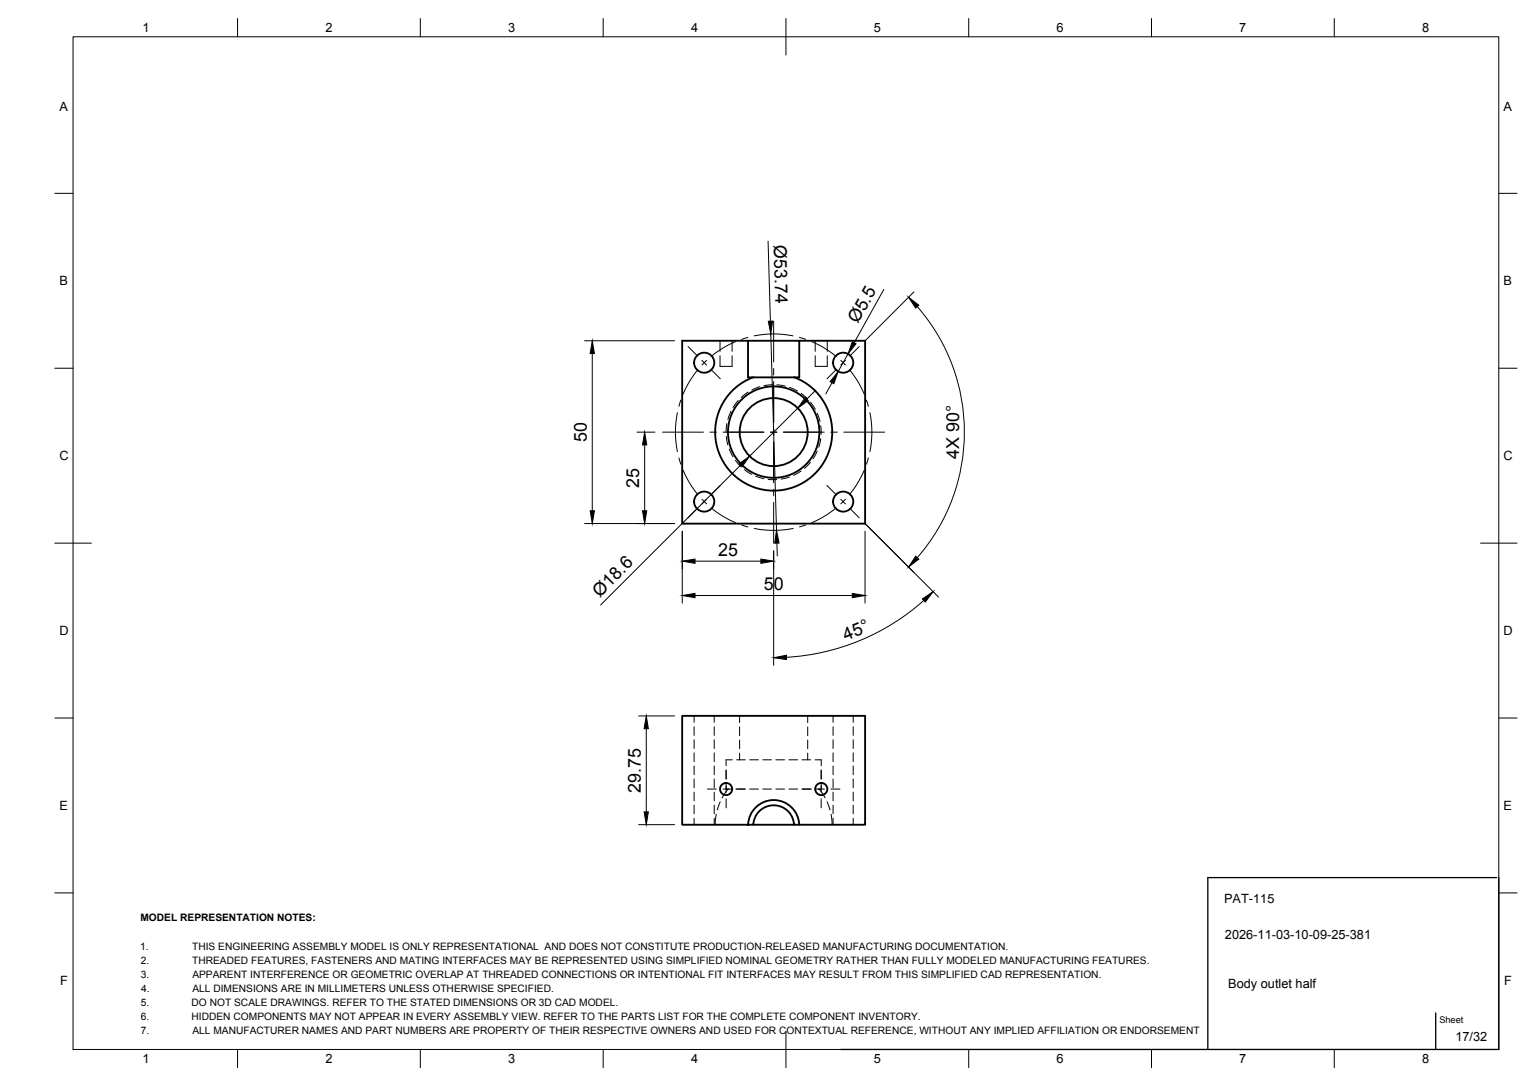
ISO-10303-21;
HEADER;
/* Generated by software containing ST-Developer
 * from STEP Tools, Inc. (www.steptools.com) 
 */

FILE_DESCRIPTION(
/* description */ ('Union bypass pipe loop'),
/* implementation_level */ '2;1');

FILE_NAME(
/* name */ 'Body outlet half.step',
/* time_stamp */ '2026-10-27T21:00:29-07:00',
/* author */ (''),
/* organization */ (''),
/* preprocessor_version */ 'ST-DEVELOPER v20.2',
/* originating_system */ 'Autodesk Translation Framework v15.17.0.0',
/* authorisation */ '');

FILE_SCHEMA (('AUTOMOTIVE_DESIGN { 1 0 10303 214 3 1 1 }'));
ENDSEC;

DATA;
#10=MECHANICAL_DESIGN_GEOMETRIC_PRESENTATION_REPRESENTATION('',(#446),#10095);
#382=SHAPE_REPRESENTATION_RELATIONSHIP('SRR','None',#10251,#414);
#414=ADVANCED_BREP_SHAPE_REPRESENTATION('',(#478),#10063);
#446=STYLED_ITEM('',(#10479),#478);
#478=MANIFOLD_SOLID_BREP('Body1',#5517);
#506=SPHERICAL_SURFACE('',#5987,1.6);
#525=FACE_BOUND('',#1213,.T.);
#526=FACE_BOUND('',#1214,.T.);
#527=FACE_BOUND('',#1218,.T.);
#528=FACE_BOUND('',#1220,.T.);
#529=FACE_BOUND('',#1222,.T.);
#530=FACE_BOUND('',#1224,.T.);
#531=FACE_BOUND('',#1225,.T.);
#532=FACE_BOUND('',#1226,.T.);
#533=FACE_BOUND('',#1227,.T.);
#534=FACE_BOUND('',#1228,.T.);
#535=FACE_BOUND('',#1231,.T.);
#536=FACE_BOUND('',#1232,.T.);
#537=FACE_BOUND('',#1233,.T.);
#538=FACE_BOUND('',#1234,.T.);
#646=PLANE('',#5955);
#647=PLANE('',#5959);
#648=PLANE('',#5975);
#649=PLANE('',#5977);
#650=PLANE('',#5984);
#651=PLANE('',#5985);
#652=PLANE('',#5989);
#653=PLANE('',#5990);
#654=PLANE('',#5991);
#655=PLANE('',#5992);
#656=PLANE('',#5993);
#856=FACE_OUTER_BOUND('',#1202,.T.);
#857=FACE_OUTER_BOUND('',#1203,.T.);
#858=FACE_OUTER_BOUND('',#1204,.T.);
#859=FACE_OUTER_BOUND('',#1205,.T.);
#860=FACE_OUTER_BOUND('',#1206,.T.);
#861=FACE_OUTER_BOUND('',#1207,.T.);
#862=FACE_OUTER_BOUND('',#1208,.T.);
#863=FACE_OUTER_BOUND('',#1209,.T.);
#864=FACE_OUTER_BOUND('',#1210,.T.);
#865=FACE_OUTER_BOUND('',#1211,.T.);
#866=FACE_OUTER_BOUND('',#1212,.T.);
#867=FACE_OUTER_BOUND('',#1215,.T.);
#868=FACE_OUTER_BOUND('',#1216,.T.);
#869=FACE_OUTER_BOUND('',#1217,.T.);
#870=FACE_OUTER_BOUND('',#1219,.T.);
#871=FACE_OUTER_BOUND('',#1221,.T.);
#872=FACE_OUTER_BOUND('',#1223,.T.);
#873=FACE_OUTER_BOUND('',#1229,.T.);
#874=FACE_OUTER_BOUND('',#1230,.T.);
#875=FACE_OUTER_BOUND('',#1235,.T.);
#876=FACE_OUTER_BOUND('',#1236,.T.);
#1202=EDGE_LOOP('',(#3830,#3831,#3832,#3833));
#1203=EDGE_LOOP('',(#3834));
#1204=EDGE_LOOP('',(#3835,#3836,#3837,#3838));
#1205=EDGE_LOOP('',(#3839));
#1206=EDGE_LOOP('',(#3840,#3841,#3842,#3843));
#1207=EDGE_LOOP('',(#3844,#3845,#3846,#3847));
#1208=EDGE_LOOP('',(#3848,#3849,#3850,#3851));
#1209=EDGE_LOOP('',(#3852,#3853,#3854,#3855));
#1210=EDGE_LOOP('',(#3856,#3857,#3858,#3859));
#1211=EDGE_LOOP('',(#3860,#3861,#3862,#3863));
#1212=EDGE_LOOP('',(#3864,#3865,#3866,#3867,#3868,#3869));
#1213=EDGE_LOOP('',(#3870));
#1214=EDGE_LOOP('',(#3871));
#1215=EDGE_LOOP('',(#3872,#3873,#3874,#3875));
#1216=EDGE_LOOP('',(#3876,#3877,#3878,#3879));
#1217=EDGE_LOOP('',(#3880));
#1218=EDGE_LOOP('',(#3881));
#1219=EDGE_LOOP('',(#3882));
#1220=EDGE_LOOP('',(#3883));
#1221=EDGE_LOOP('',(#3884,#3885));
#1222=EDGE_LOOP('',(#3886));
#1223=EDGE_LOOP('',(#3887,#3888,#3889,#3890));
#1224=EDGE_LOOP('',(#3891));
#1225=EDGE_LOOP('',(#3892));
#1226=EDGE_LOOP('',(#3893));
#1227=EDGE_LOOP('',(#3894));
#1228=EDGE_LOOP('',(#3895));
#1229=EDGE_LOOP('',(#3896,#3897,#3898,#3899));
#1230=EDGE_LOOP('',(#3900,#3901,#3902,#3903,#3904,#3905,#3906,#3907,#3908,
#3909));
#1231=EDGE_LOOP('',(#3910));
#1232=EDGE_LOOP('',(#3911));
#1233=EDGE_LOOP('',(#3912));
#1234=EDGE_LOOP('',(#3913));
#1235=EDGE_LOOP('',(#3914,#3915,#3916,#3917));
#1236=EDGE_LOOP('',(#3918,#3919,#3920,#3921));
#1648=LINE('',#8530,#2024);
#1649=LINE('',#8537,#2025);
#1650=LINE('',#8544,#2026);
#1651=LINE('',#8550,#2027);
#1652=LINE('',#8556,#2028);
#1653=LINE('',#8562,#2029);
#1654=LINE('',#8567,#2030);
#1655=LINE('',#8571,#2031);
#1656=LINE('',#8575,#2032);
#1657=LINE('',#8578,#2033);
#1658=LINE('',#8581,#2034);
#1659=LINE('',#8583,#2035);
#1660=LINE('',#8585,#2036);
#1661=LINE('',#8587,#2037);
#1662=LINE('',#8588,#2038);
#1663=LINE('',#8593,#2039);
#1664=LINE('',#8599,#2040);
#1665=LINE('',#8610,#2041);
#1666=LINE('',#8611,#2042);
#1667=LINE('',#8612,#2043);
#1668=LINE('',#8615,#2044);
#1669=LINE('',#8616,#2045);
#1670=LINE('',#8619,#2046);
#1671=LINE('',#8620,#2047);
#1672=LINE('',#8622,#2048);
#2024=VECTOR('',#6742,0.165);
#2025=VECTOR('',#6751,0.165);
#2026=VECTOR('',#6760,0.275);
#2027=VECTOR('',#6767,0.275);
#2028=VECTOR('',#6774,0.275);
#2029=VECTOR('',#6781,0.275);
#2030=VECTOR('',#6786,1.);
#2031=VECTOR('',#6789,1.);
#2032=VECTOR('',#6794,1.);
#2033=VECTOR('',#6797,1.);
#2034=VECTOR('',#6800,1.);
#2035=VECTOR('',#6801,1.);
#2036=VECTOR('',#6802,1.);
#2037=VECTOR('',#6803,1.);
#2038=VECTOR('',#6804,1.);
#2039=VECTOR('',#6809,0.93);
#2040=VECTOR('',#6816,1.3);
#2041=VECTOR('',#6831,1.);
#2042=VECTOR('',#6832,1.);
#2043=VECTOR('',#6833,1.);
#2044=VECTOR('',#6836,1.);
#2045=VECTOR('',#6837,1.);
#2046=VECTOR('',#6840,1.);
#2047=VECTOR('',#6841,1.);
#2048=VECTOR('',#6844,1.);
#2396=CIRCLE('',#5953,0.165);
#2397=CIRCLE('',#5954,0.165);
#2398=CIRCLE('',#5957,0.165);
#2399=CIRCLE('',#5958,0.165);
#2400=CIRCLE('',#5961,0.275);
#2401=CIRCLE('',#5962,0.275);
#2402=CIRCLE('',#5964,0.275);
#2403=CIRCLE('',#5965,0.275);
#2404=CIRCLE('',#5967,0.275);
#2405=CIRCLE('',#5968,0.275);
#2406=CIRCLE('',#5970,0.275);
#2407=CIRCLE('',#5971,0.275);
#2408=CIRCLE('',#5973,0.7);
#2409=CIRCLE('',#5974,0.7);
#2410=CIRCLE('',#5976,0.556776436283003);
#2411=CIRCLE('',#5979,0.93);
#2412=CIRCLE('',#5980,0.93);
#2413=CIRCLE('',#5982,1.3);
#2414=CIRCLE('',#5983,1.3);
#2415=CIRCLE('',#5986,1.24899959967968);
#2416=CIRCLE('',#5988,1.59980467557762);
#2661=VERTEX_POINT('',#8527);
#2662=VERTEX_POINT('',#8529);
#2663=VERTEX_POINT('',#8534);
#2664=VERTEX_POINT('',#8536);
#2665=VERTEX_POINT('',#8541);
#2666=VERTEX_POINT('',#8543);
#2667=VERTEX_POINT('',#8547);
#2668=VERTEX_POINT('',#8549);
#2669=VERTEX_POINT('',#8553);
#2670=VERTEX_POINT('',#8555);
#2671=VERTEX_POINT('',#8559);
#2672=VERTEX_POINT('',#8561);
#2673=VERTEX_POINT('',#8565);
#2674=VERTEX_POINT('',#8566);
#2675=VERTEX_POINT('',#8568);
#2676=VERTEX_POINT('',#8570);
#2677=VERTEX_POINT('',#8574);
#2678=VERTEX_POINT('',#8576);
#2679=VERTEX_POINT('',#8580);
#2680=VERTEX_POINT('',#8582);
#2681=VERTEX_POINT('',#8584);
#2682=VERTEX_POINT('',#8586);
#2683=VERTEX_POINT('',#8590);
#2684=VERTEX_POINT('',#8592);
#2685=VERTEX_POINT('',#8596);
#2686=VERTEX_POINT('',#8598);
#2687=VERTEX_POINT('',#8603);
#2688=VERTEX_POINT('',#8608);
#2689=VERTEX_POINT('',#8609);
#2690=VERTEX_POINT('',#8614);
#2691=VERTEX_POINT('',#8618);
#3113=EDGE_CURVE('',#2661,#2661,#2396,.T.);
#3114=EDGE_CURVE('',#2661,#2662,#1648,.T.);
#3115=EDGE_CURVE('',#2662,#2662,#2397,.T.);
#3116=EDGE_CURVE('',#2663,#2663,#2398,.T.);
#3117=EDGE_CURVE('',#2663,#2664,#1649,.T.);
#3118=EDGE_CURVE('',#2664,#2664,#2399,.T.);
#3119=EDGE_CURVE('',#2665,#2665,#2400,.T.);
#3120=EDGE_CURVE('',#2665,#2666,#1650,.T.);
#3121=EDGE_CURVE('',#2666,#2666,#2401,.T.);
#3122=EDGE_CURVE('',#2667,#2667,#2402,.T.);
#3123=EDGE_CURVE('',#2667,#2668,#1651,.T.);
#3124=EDGE_CURVE('',#2668,#2668,#2403,.T.);
#3125=EDGE_CURVE('',#2669,#2669,#2404,.T.);
#3126=EDGE_CURVE('',#2669,#2670,#1652,.T.);
#3127=EDGE_CURVE('',#2670,#2670,#2405,.T.);
#3128=EDGE_CURVE('',#2671,#2671,#2406,.T.);
#3129=EDGE_CURVE('',#2671,#2672,#1653,.T.);
#3130=EDGE_CURVE('',#2672,#2672,#2407,.T.);
#3131=EDGE_CURVE('',#2673,#2674,#1654,.T.);
#3132=EDGE_CURVE('',#2675,#2673,#2408,.T.);
#3133=EDGE_CURVE('',#2676,#2675,#1655,.T.);
#3134=EDGE_CURVE('',#2674,#2676,#2409,.T.);
#3135=EDGE_CURVE('',#2677,#2673,#1656,.T.);
#3136=EDGE_CURVE('',#2678,#2677,#2410,.T.);
#3137=EDGE_CURVE('',#2675,#2678,#1657,.T.);
#3138=EDGE_CURVE('',#2676,#2679,#1658,.T.);
#3139=EDGE_CURVE('',#2679,#2680,#1659,.T.);
#3140=EDGE_CURVE('',#2680,#2681,#1660,.T.);
#3141=EDGE_CURVE('',#2681,#2682,#1661,.T.);
#3142=EDGE_CURVE('',#2682,#2674,#1662,.T.);
#3143=EDGE_CURVE('',#2683,#2683,#2411,.T.);
#3144=EDGE_CURVE('',#2683,#2684,#1663,.T.);
#3145=EDGE_CURVE('',#2684,#2684,#2412,.T.);
#3146=EDGE_CURVE('',#2685,#2685,#2413,.T.);
#3147=EDGE_CURVE('',#2685,#2686,#1664,.T.);
#3148=EDGE_CURVE('',#2686,#2686,#2414,.T.);
#3149=EDGE_CURVE('',#2687,#2687,#2415,.T.);
#3150=EDGE_CURVE('',#2678,#2677,#2416,.T.);
#3151=EDGE_CURVE('',#2688,#2689,#1665,.T.);
#3152=EDGE_CURVE('',#2689,#2681,#1666,.T.);
#3153=EDGE_CURVE('',#2688,#2680,#1667,.T.);
#3154=EDGE_CURVE('',#2690,#2688,#1668,.T.);
#3155=EDGE_CURVE('',#2690,#2679,#1669,.T.);
#3156=EDGE_CURVE('',#2691,#2682,#1670,.T.);
#3157=EDGE_CURVE('',#2691,#2690,#1671,.T.);
#3158=EDGE_CURVE('',#2689,#2691,#1672,.T.);
#3830=ORIENTED_EDGE('',*,*,#3113,.F.);
#3831=ORIENTED_EDGE('',*,*,#3114,.T.);
#3832=ORIENTED_EDGE('',*,*,#3115,.F.);
#3833=ORIENTED_EDGE('',*,*,#3114,.F.);
#3834=ORIENTED_EDGE('',*,*,#3113,.T.);
#3835=ORIENTED_EDGE('',*,*,#3116,.F.);
#3836=ORIENTED_EDGE('',*,*,#3117,.T.);
#3837=ORIENTED_EDGE('',*,*,#3118,.F.);
#3838=ORIENTED_EDGE('',*,*,#3117,.F.);
#3839=ORIENTED_EDGE('',*,*,#3116,.T.);
#3840=ORIENTED_EDGE('',*,*,#3119,.F.);
#3841=ORIENTED_EDGE('',*,*,#3120,.T.);
#3842=ORIENTED_EDGE('',*,*,#3121,.F.);
#3843=ORIENTED_EDGE('',*,*,#3120,.F.);
#3844=ORIENTED_EDGE('',*,*,#3122,.F.);
#3845=ORIENTED_EDGE('',*,*,#3123,.T.);
#3846=ORIENTED_EDGE('',*,*,#3124,.F.);
#3847=ORIENTED_EDGE('',*,*,#3123,.F.);
#3848=ORIENTED_EDGE('',*,*,#3125,.F.);
#3849=ORIENTED_EDGE('',*,*,#3126,.T.);
#3850=ORIENTED_EDGE('',*,*,#3127,.F.);
#3851=ORIENTED_EDGE('',*,*,#3126,.F.);
#3852=ORIENTED_EDGE('',*,*,#3128,.F.);
#3853=ORIENTED_EDGE('',*,*,#3129,.T.);
#3854=ORIENTED_EDGE('',*,*,#3130,.F.);
#3855=ORIENTED_EDGE('',*,*,#3129,.F.);
#3856=ORIENTED_EDGE('',*,*,#3131,.F.);
#3857=ORIENTED_EDGE('',*,*,#3132,.F.);
#3858=ORIENTED_EDGE('',*,*,#3133,.F.);
#3859=ORIENTED_EDGE('',*,*,#3134,.F.);
#3860=ORIENTED_EDGE('',*,*,#3135,.F.);
#3861=ORIENTED_EDGE('',*,*,#3136,.F.);
#3862=ORIENTED_EDGE('',*,*,#3137,.F.);
#3863=ORIENTED_EDGE('',*,*,#3132,.T.);
#3864=ORIENTED_EDGE('',*,*,#3134,.T.);
#3865=ORIENTED_EDGE('',*,*,#3138,.T.);
#3866=ORIENTED_EDGE('',*,*,#3139,.T.);
#3867=ORIENTED_EDGE('',*,*,#3140,.T.);
#3868=ORIENTED_EDGE('',*,*,#3141,.T.);
#3869=ORIENTED_EDGE('',*,*,#3142,.T.);
#3870=ORIENTED_EDGE('',*,*,#3115,.T.);
#3871=ORIENTED_EDGE('',*,*,#3118,.T.);
#3872=ORIENTED_EDGE('',*,*,#3143,.F.);
#3873=ORIENTED_EDGE('',*,*,#3144,.T.);
#3874=ORIENTED_EDGE('',*,*,#3145,.F.);
#3875=ORIENTED_EDGE('',*,*,#3144,.F.);
#3876=ORIENTED_EDGE('',*,*,#3146,.F.);
#3877=ORIENTED_EDGE('',*,*,#3147,.T.);
#3878=ORIENTED_EDGE('',*,*,#3148,.T.);
#3879=ORIENTED_EDGE('',*,*,#3147,.F.);
#3880=ORIENTED_EDGE('',*,*,#3148,.F.);
#3881=ORIENTED_EDGE('',*,*,#3143,.T.);
#3882=ORIENTED_EDGE('',*,*,#3146,.T.);
#3883=ORIENTED_EDGE('',*,*,#3149,.F.);
#3884=ORIENTED_EDGE('',*,*,#3136,.T.);
#3885=ORIENTED_EDGE('',*,*,#3150,.F.);
#3886=ORIENTED_EDGE('',*,*,#3149,.T.);
#3887=ORIENTED_EDGE('',*,*,#3151,.T.);
#3888=ORIENTED_EDGE('',*,*,#3152,.T.);
#3889=ORIENTED_EDGE('',*,*,#3140,.F.);
#3890=ORIENTED_EDGE('',*,*,#3153,.F.);
#3891=ORIENTED_EDGE('',*,*,#3145,.T.);
#3892=ORIENTED_EDGE('',*,*,#3130,.T.);
#3893=ORIENTED_EDGE('',*,*,#3127,.T.);
#3894=ORIENTED_EDGE('',*,*,#3124,.T.);
#3895=ORIENTED_EDGE('',*,*,#3121,.T.);
#3896=ORIENTED_EDGE('',*,*,#3154,.T.);
#3897=ORIENTED_EDGE('',*,*,#3153,.T.);
#3898=ORIENTED_EDGE('',*,*,#3139,.F.);
#3899=ORIENTED_EDGE('',*,*,#3155,.F.);
#3900=ORIENTED_EDGE('',*,*,#3131,.T.);
#3901=ORIENTED_EDGE('',*,*,#3142,.F.);
#3902=ORIENTED_EDGE('',*,*,#3156,.F.);
#3903=ORIENTED_EDGE('',*,*,#3157,.T.);
#3904=ORIENTED_EDGE('',*,*,#3155,.T.);
#3905=ORIENTED_EDGE('',*,*,#3138,.F.);
#3906=ORIENTED_EDGE('',*,*,#3133,.T.);
#3907=ORIENTED_EDGE('',*,*,#3137,.T.);
#3908=ORIENTED_EDGE('',*,*,#3150,.T.);
#3909=ORIENTED_EDGE('',*,*,#3135,.T.);
#3910=ORIENTED_EDGE('',*,*,#3119,.T.);
#3911=ORIENTED_EDGE('',*,*,#3122,.T.);
#3912=ORIENTED_EDGE('',*,*,#3125,.T.);
#3913=ORIENTED_EDGE('',*,*,#3128,.T.);
#3914=ORIENTED_EDGE('',*,*,#3158,.T.);
#3915=ORIENTED_EDGE('',*,*,#3156,.T.);
#3916=ORIENTED_EDGE('',*,*,#3141,.F.);
#3917=ORIENTED_EDGE('',*,*,#3152,.F.);
#3918=ORIENTED_EDGE('',*,*,#3158,.F.);
#3919=ORIENTED_EDGE('',*,*,#3151,.F.);
#3920=ORIENTED_EDGE('',*,*,#3154,.F.);
#3921=ORIENTED_EDGE('',*,*,#3157,.F.);
#5089=CYLINDRICAL_SURFACE('',#5952,0.165);
#5090=CYLINDRICAL_SURFACE('',#5956,0.165);
#5091=CYLINDRICAL_SURFACE('',#5960,0.275);
#5092=CYLINDRICAL_SURFACE('',#5963,0.275);
#5093=CYLINDRICAL_SURFACE('',#5966,0.275);
#5094=CYLINDRICAL_SURFACE('',#5969,0.275);
#5095=CYLINDRICAL_SURFACE('',#5972,0.7);
#5096=CYLINDRICAL_SURFACE('',#5978,0.93);
#5097=CYLINDRICAL_SURFACE('',#5981,1.3);
#5205=ADVANCED_FACE('',(#856),#5089,.F.);
#5206=ADVANCED_FACE('',(#857),#646,.T.);
#5207=ADVANCED_FACE('',(#858),#5090,.F.);
#5208=ADVANCED_FACE('',(#859),#647,.T.);
#5209=ADVANCED_FACE('',(#860),#5091,.F.);
#5210=ADVANCED_FACE('',(#861),#5092,.F.);
#5211=ADVANCED_FACE('',(#862),#5093,.F.);
#5212=ADVANCED_FACE('',(#863),#5094,.F.);
#5213=ADVANCED_FACE('',(#864),#5095,.F.);
#5214=ADVANCED_FACE('',(#865),#648,.T.);
#5215=ADVANCED_FACE('',(#866,#525,#526),#649,.T.);
#5216=ADVANCED_FACE('',(#867),#5096,.F.);
#5217=ADVANCED_FACE('',(#868),#5097,.F.);
#5218=ADVANCED_FACE('',(#869,#527),#650,.F.);
#5219=ADVANCED_FACE('',(#870,#528),#651,.T.);
#5220=ADVANCED_FACE('',(#871,#529),#506,.F.);
#5221=ADVANCED_FACE('',(#872,#530,#531,#532,#533,#534),#652,.T.);
#5222=ADVANCED_FACE('',(#873),#653,.T.);
#5223=ADVANCED_FACE('',(#874,#535,#536,#537,#538),#654,.T.);
#5224=ADVANCED_FACE('',(#875),#655,.T.);
#5225=ADVANCED_FACE('',(#876),#656,.F.);
#5517=CLOSED_SHELL('',(#5205,#5206,#5207,#5208,#5209,#5210,#5211,#5212,
#5213,#5214,#5215,#5216,#5217,#5218,#5219,#5220,#5221,#5222,#5223,#5224,
#5225));
#5951=AXIS2_PLACEMENT_3D('',#8525,#6736,#6737);
#5952=AXIS2_PLACEMENT_3D('',#8526,#6738,#6739);
#5953=AXIS2_PLACEMENT_3D('',#8528,#6740,#6741);
#5954=AXIS2_PLACEMENT_3D('',#8531,#6743,#6744);
#5955=AXIS2_PLACEMENT_3D('',#8532,#6745,#6746);
#5956=AXIS2_PLACEMENT_3D('',#8533,#6747,#6748);
#5957=AXIS2_PLACEMENT_3D('',#8535,#6749,#6750);
#5958=AXIS2_PLACEMENT_3D('',#8538,#6752,#6753);
#5959=AXIS2_PLACEMENT_3D('',#8539,#6754,#6755);
#5960=AXIS2_PLACEMENT_3D('',#8540,#6756,#6757);
#5961=AXIS2_PLACEMENT_3D('',#8542,#6758,#6759);
#5962=AXIS2_PLACEMENT_3D('',#8545,#6761,#6762);
#5963=AXIS2_PLACEMENT_3D('',#8546,#6763,#6764);
#5964=AXIS2_PLACEMENT_3D('',#8548,#6765,#6766);
#5965=AXIS2_PLACEMENT_3D('',#8551,#6768,#6769);
#5966=AXIS2_PLACEMENT_3D('',#8552,#6770,#6771);
#5967=AXIS2_PLACEMENT_3D('',#8554,#6772,#6773);
#5968=AXIS2_PLACEMENT_3D('',#8557,#6775,#6776);
#5969=AXIS2_PLACEMENT_3D('',#8558,#6777,#6778);
#5970=AXIS2_PLACEMENT_3D('',#8560,#6779,#6780);
#5971=AXIS2_PLACEMENT_3D('',#8563,#6782,#6783);
#5972=AXIS2_PLACEMENT_3D('',#8564,#6784,#6785);
#5973=AXIS2_PLACEMENT_3D('',#8569,#6787,#6788);
#5974=AXIS2_PLACEMENT_3D('',#8572,#6790,#6791);
#5975=AXIS2_PLACEMENT_3D('',#8573,#6792,#6793);
#5976=AXIS2_PLACEMENT_3D('',#8577,#6795,#6796);
#5977=AXIS2_PLACEMENT_3D('',#8579,#6798,#6799);
#5978=AXIS2_PLACEMENT_3D('',#8589,#6805,#6806);
#5979=AXIS2_PLACEMENT_3D('',#8591,#6807,#6808);
#5980=AXIS2_PLACEMENT_3D('',#8594,#6810,#6811);
#5981=AXIS2_PLACEMENT_3D('',#8595,#6812,#6813);
#5982=AXIS2_PLACEMENT_3D('',#8597,#6814,#6815);
#5983=AXIS2_PLACEMENT_3D('',#8600,#6817,#6818);
#5984=AXIS2_PLACEMENT_3D('',#8601,#6819,#6820);
#5985=AXIS2_PLACEMENT_3D('',#8602,#6821,#6822);
#5986=AXIS2_PLACEMENT_3D('',#8604,#6823,#6824);
#5987=AXIS2_PLACEMENT_3D('',#8605,#6825,#6826);
#5988=AXIS2_PLACEMENT_3D('',#8606,#6827,#6828);
#5989=AXIS2_PLACEMENT_3D('',#8607,#6829,#6830);
#5990=AXIS2_PLACEMENT_3D('',#8613,#6834,#6835);
#5991=AXIS2_PLACEMENT_3D('',#8617,#6838,#6839);
#5992=AXIS2_PLACEMENT_3D('',#8621,#6842,#6843);
#5993=AXIS2_PLACEMENT_3D('',#8623,#6845,#6846);
#6736=DIRECTION('axis',(0.,0.,1.));
#6737=DIRECTION('refdir',(1.,0.,0.));
#6738=DIRECTION('center_axis',(0.,0.,1.));
#6739=DIRECTION('ref_axis',(1.,0.,0.));
#6740=DIRECTION('center_axis',(0.,0.,1.));
#6741=DIRECTION('ref_axis',(1.,0.,0.));
#6742=DIRECTION('',(0.,0.,1.));
#6743=DIRECTION('center_axis',(0.,0.,-1.));
#6744=DIRECTION('ref_axis',(1.,0.,0.));
#6745=DIRECTION('center_axis',(0.,0.,1.));
#6746=DIRECTION('ref_axis',(1.,0.,0.));
#6747=DIRECTION('center_axis',(0.,0.,1.));
#6748=DIRECTION('ref_axis',(1.,0.,0.));
#6749=DIRECTION('center_axis',(0.,0.,1.));
#6750=DIRECTION('ref_axis',(1.,0.,0.));
#6751=DIRECTION('',(0.,0.,1.));
#6752=DIRECTION('center_axis',(0.,0.,-1.));
#6753=DIRECTION('ref_axis',(1.,0.,0.));
#6754=DIRECTION('center_axis',(0.,0.,1.));
#6755=DIRECTION('ref_axis',(1.,0.,0.));
#6756=DIRECTION('center_axis',(0.,1.,0.));
#6757=DIRECTION('ref_axis',(1.,0.,0.));
#6758=DIRECTION('center_axis',(0.,1.,0.));
#6759=DIRECTION('ref_axis',(1.,0.,0.));
#6760=DIRECTION('',(0.,1.,0.));
#6761=DIRECTION('center_axis',(0.,-1.,0.));
#6762=DIRECTION('ref_axis',(1.,0.,0.));
#6763=DIRECTION('center_axis',(0.,1.,0.));
#6764=DIRECTION('ref_axis',(1.,0.,0.));
#6765=DIRECTION('center_axis',(0.,1.,0.));
#6766=DIRECTION('ref_axis',(1.,0.,0.));
#6767=DIRECTION('',(0.,1.,0.));
#6768=DIRECTION('center_axis',(0.,-1.,0.));
#6769=DIRECTION('ref_axis',(1.,0.,0.));
#6770=DIRECTION('center_axis',(0.,1.,0.));
#6771=DIRECTION('ref_axis',(1.,0.,0.));
#6772=DIRECTION('center_axis',(0.,1.,0.));
#6773=DIRECTION('ref_axis',(1.,0.,0.));
#6774=DIRECTION('',(0.,1.,0.));
#6775=DIRECTION('center_axis',(0.,-1.,0.));
#6776=DIRECTION('ref_axis',(1.,0.,0.));
#6777=DIRECTION('center_axis',(0.,1.,0.));
#6778=DIRECTION('ref_axis',(1.,0.,0.));
#6779=DIRECTION('center_axis',(0.,1.,0.));
#6780=DIRECTION('ref_axis',(1.,0.,0.));
#6781=DIRECTION('',(0.,1.,0.));
#6782=DIRECTION('center_axis',(0.,-1.,0.));
#6783=DIRECTION('ref_axis',(1.,0.,0.));
#6784=DIRECTION('center_axis',(0.,0.,1.));
#6785=DIRECTION('ref_axis',(1.,0.,0.));
#6786=DIRECTION('',(0.,0.,1.));
#6787=DIRECTION('center_axis',(0.,0.,1.));
#6788=DIRECTION('ref_axis',(1.,0.,0.));
#6789=DIRECTION('',(0.,0.,-1.));
#6790=DIRECTION('center_axis',(0.,0.,-1.));
#6791=DIRECTION('ref_axis',(1.,0.,0.));
#6792=DIRECTION('center_axis',(0.,0.,1.));
#6793=DIRECTION('ref_axis',(1.,0.,0.));
#6794=DIRECTION('',(-1.,0.,0.));
#6795=DIRECTION('center_axis',(0.,0.,1.));
#6796=DIRECTION('ref_axis',(0.,-1.,0.));
#6797=DIRECTION('',(-1.,0.,0.));
#6798=DIRECTION('center_axis',(0.,0.,1.));
#6799=DIRECTION('ref_axis',(1.,0.,0.));
#6800=DIRECTION('',(1.,0.,0.));
#6801=DIRECTION('',(0.,1.,0.));
#6802=DIRECTION('',(-1.,0.,0.));
#6803=DIRECTION('',(0.,-1.,0.));
#6804=DIRECTION('',(1.,0.,0.));
#6805=DIRECTION('center_axis',(0.,1.,0.));
#6806=DIRECTION('ref_axis',(1.,0.,0.));
#6807=DIRECTION('center_axis',(0.,1.,0.));
#6808=DIRECTION('ref_axis',(1.,0.,0.));
#6809=DIRECTION('',(0.,1.,0.));
#6810=DIRECTION('center_axis',(0.,-1.,0.));
#6811=DIRECTION('ref_axis',(1.,0.,0.));
#6812=DIRECTION('center_axis',(0.,1.,0.));
#6813=DIRECTION('ref_axis',(1.,0.,0.));
#6814=DIRECTION('center_axis',(0.,1.,0.));
#6815=DIRECTION('ref_axis',(1.,0.,0.));
#6816=DIRECTION('',(0.,1.,0.));
#6817=DIRECTION('center_axis',(0.,1.,0.));
#6818=DIRECTION('ref_axis',(1.,0.,0.));
#6819=DIRECTION('center_axis',(0.,1.,0.));
#6820=DIRECTION('ref_axis',(1.,0.,0.));
#6821=DIRECTION('center_axis',(0.,1.,0.));
#6822=DIRECTION('ref_axis',(1.,0.,0.));
#6823=DIRECTION('center_axis',(0.,1.,0.));
#6824=DIRECTION('ref_axis',(0.,0.,1.));
#6825=DIRECTION('center_axis',(6.12323399573677E-17,0.,1.));
#6826=DIRECTION('ref_axis',(1.,0.,0.));
#6827=DIRECTION('center_axis',(0.,1.,0.));
#6828=DIRECTION('ref_axis',(0.,0.,1.));
#6829=DIRECTION('center_axis',(0.,1.,0.));
#6830=DIRECTION('ref_axis',(-1.,0.,0.));
#6831=DIRECTION('',(-1.,0.,0.));
#6832=DIRECTION('',(0.,0.,1.));
#6833=DIRECTION('',(0.,0.,1.));
#6834=DIRECTION('center_axis',(1.,0.,0.));
#6835=DIRECTION('ref_axis',(0.,1.,0.));
#6836=DIRECTION('',(0.,1.,0.));
#6837=DIRECTION('',(0.,0.,1.));
#6838=DIRECTION('center_axis',(0.,-1.,0.));
#6839=DIRECTION('ref_axis',(1.,0.,0.));
#6840=DIRECTION('',(0.,0.,1.));
#6841=DIRECTION('',(1.,0.,0.));
#6842=DIRECTION('center_axis',(-1.,0.,0.));
#6843=DIRECTION('ref_axis',(0.,-1.,0.));
#6844=DIRECTION('',(0.,-1.,0.));
#6845=DIRECTION('center_axis',(0.,0.,1.));
#6846=DIRECTION('ref_axis',(1.,0.,0.));
#8525=CARTESIAN_POINT('',(0.,0.,0.));
#8526=CARTESIAN_POINT('Origin',(-1.3,1.,6.8));
#8527=CARTESIAN_POINT('',(-1.465,1.,6.8));
#8528=CARTESIAN_POINT('Origin',(-1.3,1.,6.8));
#8529=CARTESIAN_POINT('',(-1.465,1.,7.5));
#8530=CARTESIAN_POINT('',(-1.465,1.,6.8));
#8531=CARTESIAN_POINT('Origin',(-1.3,1.,7.5));
#8532=CARTESIAN_POINT('Origin',(-1.3,1.,6.8));
#8533=CARTESIAN_POINT('Origin',(1.3,1.,6.8));
#8534=CARTESIAN_POINT('',(1.135,1.,6.8));
#8535=CARTESIAN_POINT('Origin',(1.3,1.,6.8));
#8536=CARTESIAN_POINT('',(1.135,1.,7.5));
#8537=CARTESIAN_POINT('',(1.135,1.,6.8));
#8538=CARTESIAN_POINT('Origin',(1.3,1.,7.5));
#8539=CARTESIAN_POINT('Origin',(1.3,1.,6.8));
#8540=CARTESIAN_POINT('Origin',(1.9,-3.1,3.1));
#8541=CARTESIAN_POINT('',(1.625,0.0249999999999999,3.1));
#8542=CARTESIAN_POINT('Origin',(1.9,0.0249999999999999,3.1));
#8543=CARTESIAN_POINT('',(1.625,3.,3.1));
#8544=CARTESIAN_POINT('',(1.625,-3.1,3.1));
#8545=CARTESIAN_POINT('Origin',(1.9,3.,3.1));
#8546=CARTESIAN_POINT('Origin',(-1.9,-3.1,6.9));
#8547=CARTESIAN_POINT('',(-2.175,0.0249999999999999,6.9));
#8548=CARTESIAN_POINT('Origin',(-1.9,0.0249999999999999,6.9));
#8549=CARTESIAN_POINT('',(-2.175,3.,6.9));
#8550=CARTESIAN_POINT('',(-2.175,-3.1,6.9));
#8551=CARTESIAN_POINT('Origin',(-1.9,3.,6.9));
#8552=CARTESIAN_POINT('Origin',(-1.9,-3.1,3.1));
#8553=CARTESIAN_POINT('',(-2.175,0.0249999999999999,3.1));
#8554=CARTESIAN_POINT('Origin',(-1.9,0.0249999999999999,3.1));
#8555=CARTESIAN_POINT('',(-2.175,3.,3.1));
#8556=CARTESIAN_POINT('',(-2.175,-3.1,3.1));
#8557=CARTESIAN_POINT('Origin',(-1.9,3.,3.1));
#8558=CARTESIAN_POINT('Origin',(1.9,-3.1,6.9));
#8559=CARTESIAN_POINT('',(1.625,0.0249999999999999,6.9));
#8560=CARTESIAN_POINT('Origin',(1.9,0.0249999999999999,6.9));
#8561=CARTESIAN_POINT('',(1.625,3.,6.9));
#8562=CARTESIAN_POINT('',(1.625,-3.1,6.9));
#8563=CARTESIAN_POINT('Origin',(1.9,3.,6.9));
#8564=CARTESIAN_POINT('Origin',(0.,0.,6.5));
#8565=CARTESIAN_POINT('',(-0.699553428981661,0.025,6.5));
#8566=CARTESIAN_POINT('',(-0.699553428981661,0.025,7.5));
#8567=CARTESIAN_POINT('',(-0.699553428981661,0.025,6.5));
#8568=CARTESIAN_POINT('',(0.699553428981661,0.025,6.5));
#8569=CARTESIAN_POINT('Origin',(0.,0.,6.5));
#8570=CARTESIAN_POINT('',(0.699553428981661,0.025,7.5));
#8571=CARTESIAN_POINT('',(0.699553428981661,0.025,6.5));
#8572=CARTESIAN_POINT('Origin',(0.,0.,7.5));
#8573=CARTESIAN_POINT('Origin',(0.,0.,6.5));
#8574=CARTESIAN_POINT('',(-0.556214886532175,0.025,6.5));
#8575=CARTESIAN_POINT('',(-1.25,0.025,6.5));
#8576=CARTESIAN_POINT('',(0.556214886532175,0.025,6.5));
#8577=CARTESIAN_POINT('Origin',(0.,0.,6.5));
#8578=CARTESIAN_POINT('',(-1.25,0.025,6.5));
#8579=CARTESIAN_POINT('Origin',(0.,1.5125,7.5));
#8580=CARTESIAN_POINT('',(2.5,0.0249999999999999,7.5));
#8581=CARTESIAN_POINT('',(-2.5,0.025,7.5));
#8582=CARTESIAN_POINT('',(2.5,3.,7.5));
#8583=CARTESIAN_POINT('',(2.5,0.025,7.5));
#8584=CARTESIAN_POINT('',(-2.5,3.,7.5));
#8585=CARTESIAN_POINT('',(2.5,3.,7.5));
#8586=CARTESIAN_POINT('',(-2.5,0.0249999999999999,7.5));
#8587=CARTESIAN_POINT('',(-2.5,3.,7.5));
#8588=CARTESIAN_POINT('',(-2.5,0.025,7.5));
#8589=CARTESIAN_POINT('Origin',(0.,1.8,5.));
#8590=CARTESIAN_POINT('',(-0.93,1.8,5.));
#8591=CARTESIAN_POINT('Origin',(0.,1.8,5.));
#8592=CARTESIAN_POINT('',(-0.93,3.,5.));
#8593=CARTESIAN_POINT('',(-0.93,1.8,5.));
#8594=CARTESIAN_POINT('Origin',(0.,3.,5.));
#8595=CARTESIAN_POINT('Origin',(0.,1.,5.));
#8596=CARTESIAN_POINT('',(-1.3,1.,5.));
#8597=CARTESIAN_POINT('Origin',(0.,1.,5.));
#8598=CARTESIAN_POINT('',(-1.3,1.8,5.));
#8599=CARTESIAN_POINT('',(-1.3,1.,5.));
#8600=CARTESIAN_POINT('Origin',(0.,1.8,5.));
#8601=CARTESIAN_POINT('Origin',(0.,1.8,5.));
#8602=CARTESIAN_POINT('Origin',(0.,1.,5.));
#8603=CARTESIAN_POINT('',(-1.52958336188405E-16,1.,3.75100040032032));
#8604=CARTESIAN_POINT('Origin',(0.,1.,5.));
#8605=CARTESIAN_POINT('Origin',(0.,0.,5.));
#8606=CARTESIAN_POINT('Origin',(0.,0.025,5.));
#8607=CARTESIAN_POINT('Origin',(2.5,3.,2.5));
#8608=CARTESIAN_POINT('',(2.5,3.,2.5));
#8609=CARTESIAN_POINT('',(-2.5,3.,2.5));
#8610=CARTESIAN_POINT('',(2.5,3.,2.5));
#8611=CARTESIAN_POINT('',(-2.5,3.,2.5));
#8612=CARTESIAN_POINT('',(2.5,3.,2.5));
#8613=CARTESIAN_POINT('Origin',(2.5,0.025,2.5));
#8614=CARTESIAN_POINT('',(2.5,0.025,2.5));
#8615=CARTESIAN_POINT('',(2.5,0.025,2.5));
#8616=CARTESIAN_POINT('',(2.5,0.025,2.5));
#8617=CARTESIAN_POINT('Origin',(-2.5,0.025,2.5));
#8618=CARTESIAN_POINT('',(-2.5,0.0249999999999999,2.5));
#8619=CARTESIAN_POINT('',(-2.5,0.0249999999999999,2.5));
#8620=CARTESIAN_POINT('',(-2.5,0.025,2.5));
#8621=CARTESIAN_POINT('Origin',(-2.5,3.,2.5));
#8622=CARTESIAN_POINT('',(-2.5,3.,2.5));
#8623=CARTESIAN_POINT('Origin',(0.,1.5125,2.5));
#10026=UNCERTAINTY_MEASURE_WITH_UNIT(LENGTH_MEASURE(0.001),#10096,
'DISTANCE_ACCURACY_VALUE',
'Maximum model space distance between geometric entities at asserted c
onnectivities');
#10058=UNCERTAINTY_MEASURE_WITH_UNIT(LENGTH_MEASURE(0.001),#10096,
'DISTANCE_ACCURACY_VALUE',
'Maximum model space distance between geometric entities at asserted c
onnectivities');
#10063=(
GEOMETRIC_REPRESENTATION_CONTEXT(3)
GLOBAL_UNCERTAINTY_ASSIGNED_CONTEXT((#10026))
GLOBAL_UNIT_ASSIGNED_CONTEXT((#10096,#10098,#10099))
REPRESENTATION_CONTEXT('','3D')
);
#10095=(
GEOMETRIC_REPRESENTATION_CONTEXT(3)
GLOBAL_UNCERTAINTY_ASSIGNED_CONTEXT((#10058))
GLOBAL_UNIT_ASSIGNED_CONTEXT((#10096,#10098,#10099))
REPRESENTATION_CONTEXT('','3D')
);
#10096=(
LENGTH_UNIT()
NAMED_UNIT(*)
SI_UNIT(.CENTI.,.METRE.)
);
#10098=(
NAMED_UNIT(*)
PLANE_ANGLE_UNIT()
SI_UNIT($,.RADIAN.)
);
#10099=(
NAMED_UNIT(*)
SI_UNIT($,.STERADIAN.)
SOLID_ANGLE_UNIT()
);
#10104=SHAPE_DEFINITION_REPRESENTATION(#10140,#10251);
#10140=PRODUCT_DEFINITION_SHAPE('',$,#10288);
#10251=SHAPE_REPRESENTATION('',(#5951),#10063);
#10283=PRODUCT_DEFINITION_CONTEXT('part definition',#10393,'design');
#10288=PRODUCT_DEFINITION('Body outlet half','Body outlet half',#10324,
#10283);
#10324=PRODUCT_DEFINITION_FORMATION('',$,#10399);
#10393=APPLICATION_CONTEXT(
'Core Data for Automotive Mechanical Design Process');
#10394=PRODUCT_CONTEXT('part definition',#10393,'mechanical');
#10399=PRODUCT('Body outlet half','Body outlet half','Body outlet half',
(#10394));
#10473=COLOUR_RGB('Dark Blue',0.08,0.2,0.34);
#10474=FILL_AREA_STYLE_COLOUR('',#10473);
#10475=FILL_AREA_STYLE('',(#10474));
#10476=SURFACE_STYLE_FILL_AREA(#10475);
#10477=SURFACE_SIDE_STYLE('',(#10476));
#10478=SURFACE_STYLE_USAGE(.BOTH.,#10477);
#10479=PRESENTATION_STYLE_ASSIGNMENT((#10478));
ENDSEC;
END-ISO-10303-21;
